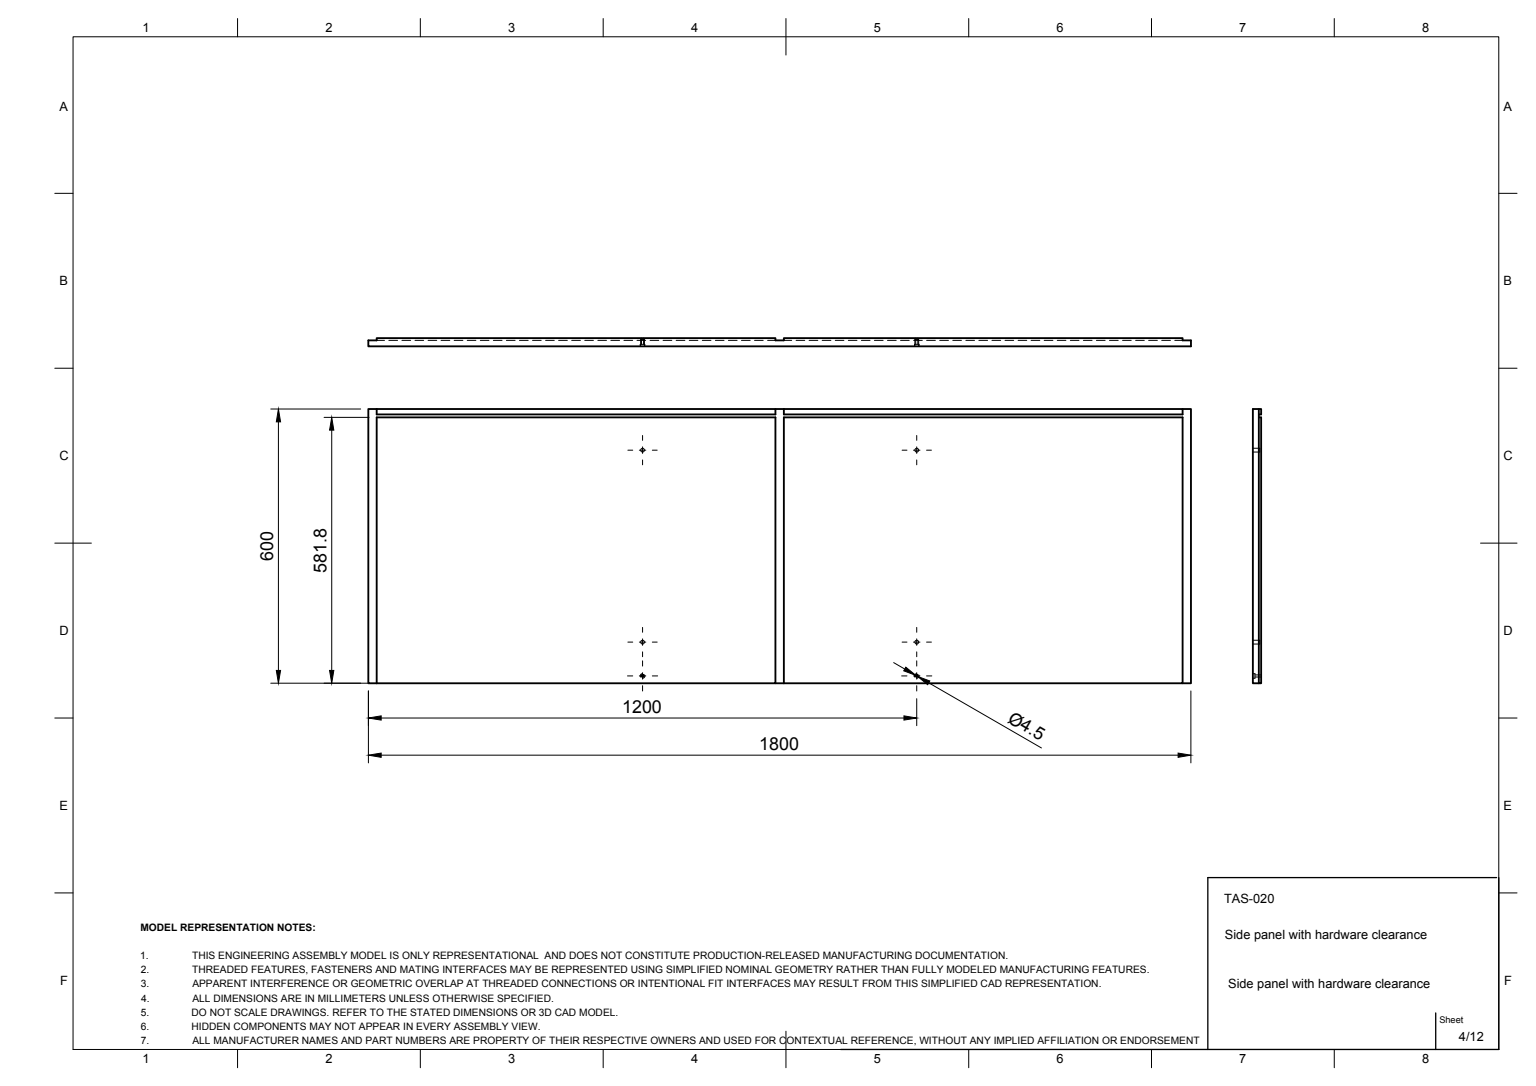
ISO-10303-21;
HEADER;
/* Generated by software containing ST-Developer
 * from STEP Tools, Inc. (www.steptools.com) 
 */

FILE_DESCRIPTION(
/* description */ (''),
/* implementation_level */ '2;1');

FILE_NAME(
/* name */ 'Side panel with hardware clearance.step',
/* time_stamp */ '2026-11-15T17:46:57-08:00',
/* author */ (''),
/* organization */ (''),
/* preprocessor_version */ 'ST-DEVELOPER v20.2',
/* originating_system */ 'Autodesk Translation Framework v15.17.0.0',
/* authorisation */ '');

FILE_SCHEMA (('AUTOMOTIVE_DESIGN { 1 0 10303 214 3 1 1 }'));
ENDSEC;

DATA;
#10=MECHANICAL_DESIGN_GEOMETRIC_PRESENTATION_REPRESENTATION('',(#375),#12963);
#351=SHAPE_REPRESENTATION_RELATIONSHIP('SRR','None',#13035,#363);
#363=ADVANCED_BREP_SHAPE_REPRESENTATION('',(#387),#12951);
#375=STYLED_ITEM('',(#13104),#387);
#387=MANIFOLD_SOLID_BREP('Body1',#4809);
#399=FACE_BOUND('',#830,.T.);
#400=FACE_BOUND('',#833,.T.);
#401=FACE_BOUND('',#852,.T.);
#402=FACE_BOUND('',#859,.T.);
#403=FACE_BOUND('',#867,.T.);
#404=FACE_BOUND('',#868,.T.);
#405=FACE_BOUND('',#869,.T.);
#406=FACE_BOUND('',#870,.T.);
#407=FACE_BOUND('',#871,.T.);
#408=FACE_BOUND('',#872,.T.);
#441=PLANE('',#4959);
#442=PLANE('',#4964);
#443=PLANE('',#4969);
#444=PLANE('',#4973);
#445=PLANE('',#4977);
#446=PLANE('',#4981);
#447=PLANE('',#4986);
#448=PLANE('',#4987);
#449=PLANE('',#4988);
#450=PLANE('',#4989);
#451=PLANE('',#4990);
#452=PLANE('',#4991);
#453=PLANE('',#4992);
#454=PLANE('',#4993);
#455=PLANE('',#4994);
#456=PLANE('',#4995);
#457=PLANE('',#4996);
#458=PLANE('',#4997);
#459=PLANE('',#4998);
#460=PLANE('',#4999);
#461=PLANE('',#5000);
#462=PLANE('',#5001);
#463=PLANE('',#5002);
#464=PLANE('',#5003);
#465=PLANE('',#5004);
#466=PLANE('',#5005);
#467=PLANE('',#5006);
#468=PLANE('',#5007);
#572=FACE_OUTER_BOUND('',#828,.T.);
#573=FACE_OUTER_BOUND('',#829,.T.);
#574=FACE_OUTER_BOUND('',#831,.T.);
#575=FACE_OUTER_BOUND('',#832,.T.);
#576=FACE_OUTER_BOUND('',#834,.T.);
#577=FACE_OUTER_BOUND('',#835,.T.);
#578=FACE_OUTER_BOUND('',#836,.T.);
#579=FACE_OUTER_BOUND('',#837,.T.);
#580=FACE_OUTER_BOUND('',#838,.T.);
#581=FACE_OUTER_BOUND('',#839,.T.);
#582=FACE_OUTER_BOUND('',#840,.T.);
#583=FACE_OUTER_BOUND('',#841,.T.);
#584=FACE_OUTER_BOUND('',#842,.T.);
#585=FACE_OUTER_BOUND('',#843,.T.);
#586=FACE_OUTER_BOUND('',#844,.T.);
#587=FACE_OUTER_BOUND('',#845,.T.);
#588=FACE_OUTER_BOUND('',#846,.T.);
#589=FACE_OUTER_BOUND('',#847,.T.);
#590=FACE_OUTER_BOUND('',#848,.T.);
#591=FACE_OUTER_BOUND('',#849,.T.);
#592=FACE_OUTER_BOUND('',#850,.T.);
#593=FACE_OUTER_BOUND('',#851,.T.);
#594=FACE_OUTER_BOUND('',#853,.T.);
#595=FACE_OUTER_BOUND('',#854,.T.);
#596=FACE_OUTER_BOUND('',#855,.T.);
#597=FACE_OUTER_BOUND('',#856,.T.);
#598=FACE_OUTER_BOUND('',#857,.T.);
#599=FACE_OUTER_BOUND('',#858,.T.);
#600=FACE_OUTER_BOUND('',#860,.T.);
#601=FACE_OUTER_BOUND('',#861,.T.);
#602=FACE_OUTER_BOUND('',#862,.T.);
#603=FACE_OUTER_BOUND('',#863,.T.);
#604=FACE_OUTER_BOUND('',#864,.T.);
#605=FACE_OUTER_BOUND('',#865,.T.);
#606=FACE_OUTER_BOUND('',#866,.T.);
#607=FACE_OUTER_BOUND('',#873,.T.);
#828=EDGE_LOOP('',(#3112,#3113,#3114,#3115));
#829=EDGE_LOOP('',(#3116));
#830=EDGE_LOOP('',(#3117));
#831=EDGE_LOOP('',(#3118,#3119,#3120,#3121));
#832=EDGE_LOOP('',(#3122));
#833=EDGE_LOOP('',(#3123));
#834=EDGE_LOOP('',(#3124,#3125,#3126,#3127));
#835=EDGE_LOOP('',(#3128));
#836=EDGE_LOOP('',(#3129,#3130,#3131,#3132));
#837=EDGE_LOOP('',(#3133));
#838=EDGE_LOOP('',(#3134,#3135,#3136,#3137));
#839=EDGE_LOOP('',(#3138));
#840=EDGE_LOOP('',(#3139,#3140,#3141,#3142));
#841=EDGE_LOOP('',(#3143));
#842=EDGE_LOOP('',(#3144,#3145,#3146,#3147));
#843=EDGE_LOOP('',(#3148,#3149,#3150,#3151));
#844=EDGE_LOOP('',(#3152,#3153,#3154,#3155));
#845=EDGE_LOOP('',(#3156,#3157,#3158,#3159));
#846=EDGE_LOOP('',(#3160,#3161,#3162,#3163));
#847=EDGE_LOOP('',(#3164,#3165,#3166,#3167));
#848=EDGE_LOOP('',(#3168,#3169,#3170,#3171,#3172,#3173,#3174,#3175,#3176,
#3177,#3178,#3179,#3180,#3181,#3182,#3183,#3184,#3185,#3186,#3187));
#849=EDGE_LOOP('',(#3188,#3189,#3190,#3191));
#850=EDGE_LOOP('',(#3192,#3193,#3194,#3195));
#851=EDGE_LOOP('',(#3196,#3197,#3198,#3199));
#852=EDGE_LOOP('',(#3200));
#853=EDGE_LOOP('',(#3201,#3202,#3203,#3204));
#854=EDGE_LOOP('',(#3205,#3206,#3207,#3208));
#855=EDGE_LOOP('',(#3209,#3210,#3211,#3212));
#856=EDGE_LOOP('',(#3213,#3214,#3215,#3216));
#857=EDGE_LOOP('',(#3217,#3218,#3219,#3220));
#858=EDGE_LOOP('',(#3221,#3222,#3223,#3224));
#859=EDGE_LOOP('',(#3225));
#860=EDGE_LOOP('',(#3226,#3227,#3228,#3229));
#861=EDGE_LOOP('',(#3230,#3231,#3232,#3233));
#862=EDGE_LOOP('',(#3234,#3235,#3236,#3237));
#863=EDGE_LOOP('',(#3238,#3239,#3240,#3241,#3242,#3243,#3244,#3245,#3246,
#3247,#3248,#3249));
#864=EDGE_LOOP('',(#3250,#3251,#3252,#3253));
#865=EDGE_LOOP('',(#3254,#3255,#3256,#3257,#3258,#3259,#3260,#3261,#3262,
#3263,#3264,#3265));
#866=EDGE_LOOP('',(#3266,#3267,#3268,#3269));
#867=EDGE_LOOP('',(#3270));
#868=EDGE_LOOP('',(#3271));
#869=EDGE_LOOP('',(#3272));
#870=EDGE_LOOP('',(#3273));
#871=EDGE_LOOP('',(#3274));
#872=EDGE_LOOP('',(#3275));
#873=EDGE_LOOP('',(#3276,#3277,#3278,#3279));
#1126=LINE('',#6523,#1528);
#1127=LINE('',#6532,#1529);
#1128=LINE('',#6541,#1530);
#1129=LINE('',#6548,#1531);
#1130=LINE('',#6555,#1532);
#1131=LINE('',#6562,#1533);
#1132=LINE('',#6568,#1534);
#1133=LINE('',#6572,#1535);
#1134=LINE('',#6576,#1536);
#1135=LINE('',#6578,#1537);
#1136=LINE('',#6580,#1538);
#1137=LINE('',#6581,#1539);
#1138=LINE('',#6585,#1540);
#1139=LINE('',#6587,#1541);
#1140=LINE('',#6589,#1542);
#1141=LINE('',#6590,#1543);
#1142=LINE('',#6594,#1544);
#1143=LINE('',#6596,#1545);
#1144=LINE('',#6598,#1546);
#1145=LINE('',#6599,#1547);
#1146=LINE('',#6603,#1548);
#1147=LINE('',#6605,#1549);
#1148=LINE('',#6607,#1550);
#1149=LINE('',#6608,#1551);
#1150=LINE('',#6611,#1552);
#1151=LINE('',#6613,#1553);
#1152=LINE('',#6615,#1554);
#1153=LINE('',#6617,#1555);
#1154=LINE('',#6618,#1556);
#1155=LINE('',#6620,#1557);
#1156=LINE('',#6622,#1558);
#1157=LINE('',#6623,#1559);
#1158=LINE('',#6625,#1560);
#1159=LINE('',#6627,#1561);
#1160=LINE('',#6629,#1562);
#1161=LINE('',#6631,#1563);
#1162=LINE('',#6632,#1564);
#1163=LINE('',#6634,#1565);
#1164=LINE('',#6636,#1566);
#1165=LINE('',#6637,#1567);
#1166=LINE('',#6640,#1568);
#1167=LINE('',#6641,#1569);
#1168=LINE('',#6644,#1570);
#1169=LINE('',#6645,#1571);
#1170=LINE('',#6648,#1572);
#1171=LINE('',#6649,#1573);
#1172=LINE('',#6652,#1574);
#1173=LINE('',#6653,#1575);
#1174=LINE('',#6655,#1576);
#1175=LINE('',#6657,#1577);
#1176=LINE('',#6660,#1578);
#1177=LINE('',#6661,#1579);
#1178=LINE('',#6664,#1580);
#1179=LINE('',#6665,#1581);
#1180=LINE('',#6668,#1582);
#1181=LINE('',#6669,#1583);
#1182=LINE('',#6672,#1584);
#1183=LINE('',#6673,#1585);
#1184=LINE('',#6675,#1586);
#1185=LINE('',#6677,#1587);
#1186=LINE('',#6680,#1588);
#1187=LINE('',#6682,#1589);
#1188=LINE('',#6683,#1590);
#1189=LINE('',#6686,#1591);
#1190=LINE('',#6687,#1592);
#1191=LINE('',#6690,#1593);
#1192=LINE('',#6691,#1594);
#1193=LINE('',#6693,#1595);
#1528=VECTOR('',#5349,0.5);
#1529=VECTOR('',#5360,0.5);
#1530=VECTOR('',#5371,0.409999999999997);
#1531=VECTOR('',#5380,0.409999999999997);
#1532=VECTOR('',#5389,0.409999999999997);
#1533=VECTOR('',#5398,0.409999999999997);
#1534=VECTOR('',#5407,0.225000000000001);
#1535=VECTOR('',#5412,0.224999999999994);
#1536=VECTOR('',#5415,1.);
#1537=VECTOR('',#5416,1.);
#1538=VECTOR('',#5417,1.);
#1539=VECTOR('',#5418,1.);
#1540=VECTOR('',#5421,1.);
#1541=VECTOR('',#5422,1.);
#1542=VECTOR('',#5423,1.);
#1543=VECTOR('',#5424,1.);
#1544=VECTOR('',#5427,1.);
#1545=VECTOR('',#5428,1.);
#1546=VECTOR('',#5429,1.);
#1547=VECTOR('',#5430,1.);
#1548=VECTOR('',#5433,1.);
#1549=VECTOR('',#5434,1.);
#1550=VECTOR('',#5435,1.);
#1551=VECTOR('',#5436,1.);
#1552=VECTOR('',#5439,1.);
#1553=VECTOR('',#5440,1.);
#1554=VECTOR('',#5441,1.);
#1555=VECTOR('',#5442,1.);
#1556=VECTOR('',#5443,1.);
#1557=VECTOR('',#5444,1.);
#1558=VECTOR('',#5445,1.);
#1559=VECTOR('',#5446,1.);
#1560=VECTOR('',#5447,1.);
#1561=VECTOR('',#5448,1.);
#1562=VECTOR('',#5449,1.);
#1563=VECTOR('',#5450,1.);
#1564=VECTOR('',#5451,1.);
#1565=VECTOR('',#5452,1.);
#1566=VECTOR('',#5453,1.);
#1567=VECTOR('',#5454,1.);
#1568=VECTOR('',#5457,1.);
#1569=VECTOR('',#5458,1.);
#1570=VECTOR('',#5461,1.);
#1571=VECTOR('',#5462,1.);
#1572=VECTOR('',#5465,1.);
#1573=VECTOR('',#5466,1.);
#1574=VECTOR('',#5469,1.);
#1575=VECTOR('',#5470,1.);
#1576=VECTOR('',#5473,1.);
#1577=VECTOR('',#5476,1.);
#1578=VECTOR('',#5479,1.);
#1579=VECTOR('',#5480,1.);
#1580=VECTOR('',#5483,1.);
#1581=VECTOR('',#5484,1.);
#1582=VECTOR('',#5487,1.);
#1583=VECTOR('',#5488,1.);
#1584=VECTOR('',#5491,1.);
#1585=VECTOR('',#5492,1.);
#1586=VECTOR('',#5495,1.);
#1587=VECTOR('',#5498,1.);
#1588=VECTOR('',#5501,1.);
#1589=VECTOR('',#5502,1.);
#1590=VECTOR('',#5503,1.);
#1591=VECTOR('',#5506,1.);
#1592=VECTOR('',#5507,1.);
#1593=VECTOR('',#5510,1.);
#1594=VECTOR('',#5511,1.);
#1595=VECTOR('',#5514,1.);
#1930=CIRCLE('',#4957,0.5);
#1931=CIRCLE('',#4958,0.5);
#1932=CIRCLE('',#4960,0.225000000000001);
#1933=CIRCLE('',#4962,0.5);
#1934=CIRCLE('',#4963,0.5);
#1935=CIRCLE('',#4965,0.224999999999994);
#1936=CIRCLE('',#4967,0.409999999999997);
#1937=CIRCLE('',#4968,0.409999999999997);
#1938=CIRCLE('',#4971,0.409999999999997);
#1939=CIRCLE('',#4972,0.409999999999997);
#1940=CIRCLE('',#4975,0.409999999999997);
#1941=CIRCLE('',#4976,0.409999999999997);
#1942=CIRCLE('',#4979,0.409999999999997);
#1943=CIRCLE('',#4980,0.409999999999997);
#1944=CIRCLE('',#4983,0.225000000000001);
#1945=CIRCLE('',#4985,0.224999999999994);
#2012=VERTEX_POINT('',#6520);
#2013=VERTEX_POINT('',#6522);
#2014=VERTEX_POINT('',#6526);
#2015=VERTEX_POINT('',#6529);
#2016=VERTEX_POINT('',#6531);
#2017=VERTEX_POINT('',#6535);
#2018=VERTEX_POINT('',#6538);
#2019=VERTEX_POINT('',#6540);
#2020=VERTEX_POINT('',#6545);
#2021=VERTEX_POINT('',#6547);
#2022=VERTEX_POINT('',#6552);
#2023=VERTEX_POINT('',#6554);
#2024=VERTEX_POINT('',#6559);
#2025=VERTEX_POINT('',#6561);
#2026=VERTEX_POINT('',#6566);
#2027=VERTEX_POINT('',#6570);
#2028=VERTEX_POINT('',#6574);
#2029=VERTEX_POINT('',#6575);
#2030=VERTEX_POINT('',#6577);
#2031=VERTEX_POINT('',#6579);
#2032=VERTEX_POINT('',#6583);
#2033=VERTEX_POINT('',#6584);
#2034=VERTEX_POINT('',#6586);
#2035=VERTEX_POINT('',#6588);
#2036=VERTEX_POINT('',#6592);
#2037=VERTEX_POINT('',#6593);
#2038=VERTEX_POINT('',#6595);
#2039=VERTEX_POINT('',#6597);
#2040=VERTEX_POINT('',#6601);
#2041=VERTEX_POINT('',#6602);
#2042=VERTEX_POINT('',#6604);
#2043=VERTEX_POINT('',#6606);
#2044=VERTEX_POINT('',#6610);
#2045=VERTEX_POINT('',#6612);
#2046=VERTEX_POINT('',#6614);
#2047=VERTEX_POINT('',#6616);
#2048=VERTEX_POINT('',#6619);
#2049=VERTEX_POINT('',#6621);
#2050=VERTEX_POINT('',#6624);
#2051=VERTEX_POINT('',#6626);
#2052=VERTEX_POINT('',#6628);
#2053=VERTEX_POINT('',#6630);
#2054=VERTEX_POINT('',#6633);
#2055=VERTEX_POINT('',#6635);
#2056=VERTEX_POINT('',#6639);
#2057=VERTEX_POINT('',#6643);
#2058=VERTEX_POINT('',#6647);
#2059=VERTEX_POINT('',#6651);
#2060=VERTEX_POINT('',#6659);
#2061=VERTEX_POINT('',#6663);
#2062=VERTEX_POINT('',#6667);
#2063=VERTEX_POINT('',#6671);
#2064=VERTEX_POINT('',#6679);
#2065=VERTEX_POINT('',#6681);
#2066=VERTEX_POINT('',#6685);
#2067=VERTEX_POINT('',#6689);
#2452=EDGE_CURVE('',#2012,#2012,#1930,.T.);
#2453=EDGE_CURVE('',#2012,#2013,#1126,.T.);
#2454=EDGE_CURVE('',#2013,#2013,#1931,.T.);
#2455=EDGE_CURVE('',#2014,#2014,#1932,.T.);
#2456=EDGE_CURVE('',#2015,#2015,#1933,.T.);
#2457=EDGE_CURVE('',#2015,#2016,#1127,.T.);
#2458=EDGE_CURVE('',#2016,#2016,#1934,.T.);
#2459=EDGE_CURVE('',#2017,#2017,#1935,.T.);
#2460=EDGE_CURVE('',#2018,#2018,#1936,.T.);
#2461=EDGE_CURVE('',#2018,#2019,#1128,.T.);
#2462=EDGE_CURVE('',#2019,#2019,#1937,.T.);
#2463=EDGE_CURVE('',#2020,#2020,#1938,.T.);
#2464=EDGE_CURVE('',#2020,#2021,#1129,.T.);
#2465=EDGE_CURVE('',#2021,#2021,#1939,.T.);
#2466=EDGE_CURVE('',#2022,#2022,#1940,.T.);
#2467=EDGE_CURVE('',#2022,#2023,#1130,.T.);
#2468=EDGE_CURVE('',#2023,#2023,#1941,.T.);
#2469=EDGE_CURVE('',#2024,#2024,#1942,.T.);
#2470=EDGE_CURVE('',#2024,#2025,#1131,.T.);
#2471=EDGE_CURVE('',#2025,#2025,#1943,.T.);
#2472=EDGE_CURVE('',#2026,#2026,#1944,.T.);
#2473=EDGE_CURVE('',#2026,#2014,#1132,.T.);
#2474=EDGE_CURVE('',#2027,#2027,#1945,.T.);
#2475=EDGE_CURVE('',#2027,#2017,#1133,.T.);
#2476=EDGE_CURVE('',#2028,#2029,#1134,.T.);
#2477=EDGE_CURVE('',#2030,#2028,#1135,.T.);
#2478=EDGE_CURVE('',#2031,#2030,#1136,.T.);
#2479=EDGE_CURVE('',#2029,#2031,#1137,.T.);
#2480=EDGE_CURVE('',#2032,#2033,#1138,.T.);
#2481=EDGE_CURVE('',#2034,#2032,#1139,.T.);
#2482=EDGE_CURVE('',#2035,#2034,#1140,.T.);
#2483=EDGE_CURVE('',#2033,#2035,#1141,.T.);
#2484=EDGE_CURVE('',#2036,#2037,#1142,.T.);
#2485=EDGE_CURVE('',#2038,#2036,#1143,.T.);
#2486=EDGE_CURVE('',#2039,#2038,#1144,.T.);
#2487=EDGE_CURVE('',#2039,#2037,#1145,.T.);
#2488=EDGE_CURVE('',#2040,#2041,#1146,.T.);
#2489=EDGE_CURVE('',#2042,#2040,#1147,.T.);
#2490=EDGE_CURVE('',#2043,#2042,#1148,.T.);
#2491=EDGE_CURVE('',#2043,#2041,#1149,.T.);
#2492=EDGE_CURVE('',#2044,#2032,#1150,.T.);
#2493=EDGE_CURVE('',#2045,#2044,#1151,.T.);
#2494=EDGE_CURVE('',#2046,#2045,#1152,.T.);
#2495=EDGE_CURVE('',#2047,#2046,#1153,.T.);
#2496=EDGE_CURVE('',#2041,#2047,#1154,.T.);
#2497=EDGE_CURVE('',#2043,#2048,#1155,.T.);
#2498=EDGE_CURVE('',#2049,#2048,#1156,.T.);
#2499=EDGE_CURVE('',#2037,#2049,#1157,.T.);
#2500=EDGE_CURVE('',#2039,#2050,#1158,.T.);
#2501=EDGE_CURVE('',#2051,#2050,#1159,.T.);
#2502=EDGE_CURVE('',#2052,#2051,#1160,.T.);
#2503=EDGE_CURVE('',#2053,#2052,#1161,.T.);
#2504=EDGE_CURVE('',#2053,#2030,#1162,.T.);
#2505=EDGE_CURVE('',#2054,#2028,#1163,.T.);
#2506=EDGE_CURVE('',#2055,#2054,#1164,.T.);
#2507=EDGE_CURVE('',#2055,#2034,#1165,.T.);
#2508=EDGE_CURVE('',#2056,#2047,#1166,.T.);
#2509=EDGE_CURVE('',#2040,#2056,#1167,.T.);
#2510=EDGE_CURVE('',#2057,#2033,#1168,.T.);
#2511=EDGE_CURVE('',#2044,#2057,#1169,.T.);
#2512=EDGE_CURVE('',#2058,#2056,#1170,.T.);
#2513=EDGE_CURVE('',#2058,#2042,#1171,.T.);
#2514=EDGE_CURVE('',#2035,#2059,#1172,.T.);
#2515=EDGE_CURVE('',#2059,#2057,#1173,.T.);
#2516=EDGE_CURVE('',#2048,#2058,#1174,.T.);
#2517=EDGE_CURVE('',#2059,#2055,#1175,.T.);
#2518=EDGE_CURVE('',#2060,#2049,#1176,.T.);
#2519=EDGE_CURVE('',#2036,#2060,#1177,.T.);
#2520=EDGE_CURVE('',#2061,#2029,#1178,.T.);
#2521=EDGE_CURVE('',#2054,#2061,#1179,.T.);
#2522=EDGE_CURVE('',#2062,#2060,#1180,.T.);
#2523=EDGE_CURVE('',#2062,#2038,#1181,.T.);
#2524=EDGE_CURVE('',#2031,#2063,#1182,.T.);
#2525=EDGE_CURVE('',#2063,#2061,#1183,.T.);
#2526=EDGE_CURVE('',#2050,#2062,#1184,.T.);
#2527=EDGE_CURVE('',#2063,#2053,#1185,.T.);
#2528=EDGE_CURVE('',#2052,#2064,#1186,.T.);
#2529=EDGE_CURVE('',#2064,#2065,#1187,.T.);
#2530=EDGE_CURVE('',#2045,#2065,#1188,.T.);
#2531=EDGE_CURVE('',#2066,#2051,#1189,.T.);
#2532=EDGE_CURVE('',#2064,#2066,#1190,.T.);
#2533=EDGE_CURVE('',#2067,#2046,#1191,.T.);
#2534=EDGE_CURVE('',#2066,#2067,#1192,.T.);
#2535=EDGE_CURVE('',#2065,#2067,#1193,.T.);
#3112=ORIENTED_EDGE('',*,*,#2452,.F.);
#3113=ORIENTED_EDGE('',*,*,#2453,.T.);
#3114=ORIENTED_EDGE('',*,*,#2454,.T.);
#3115=ORIENTED_EDGE('',*,*,#2453,.F.);
#3116=ORIENTED_EDGE('',*,*,#2454,.F.);
#3117=ORIENTED_EDGE('',*,*,#2455,.F.);
#3118=ORIENTED_EDGE('',*,*,#2456,.F.);
#3119=ORIENTED_EDGE('',*,*,#2457,.T.);
#3120=ORIENTED_EDGE('',*,*,#2458,.T.);
#3121=ORIENTED_EDGE('',*,*,#2457,.F.);
#3122=ORIENTED_EDGE('',*,*,#2458,.F.);
#3123=ORIENTED_EDGE('',*,*,#2459,.F.);
#3124=ORIENTED_EDGE('',*,*,#2460,.F.);
#3125=ORIENTED_EDGE('',*,*,#2461,.T.);
#3126=ORIENTED_EDGE('',*,*,#2462,.T.);
#3127=ORIENTED_EDGE('',*,*,#2461,.F.);
#3128=ORIENTED_EDGE('',*,*,#2462,.F.);
#3129=ORIENTED_EDGE('',*,*,#2463,.F.);
#3130=ORIENTED_EDGE('',*,*,#2464,.T.);
#3131=ORIENTED_EDGE('',*,*,#2465,.T.);
#3132=ORIENTED_EDGE('',*,*,#2464,.F.);
#3133=ORIENTED_EDGE('',*,*,#2465,.F.);
#3134=ORIENTED_EDGE('',*,*,#2466,.F.);
#3135=ORIENTED_EDGE('',*,*,#2467,.T.);
#3136=ORIENTED_EDGE('',*,*,#2468,.T.);
#3137=ORIENTED_EDGE('',*,*,#2467,.F.);
#3138=ORIENTED_EDGE('',*,*,#2468,.F.);
#3139=ORIENTED_EDGE('',*,*,#2469,.F.);
#3140=ORIENTED_EDGE('',*,*,#2470,.T.);
#3141=ORIENTED_EDGE('',*,*,#2471,.T.);
#3142=ORIENTED_EDGE('',*,*,#2470,.F.);
#3143=ORIENTED_EDGE('',*,*,#2471,.F.);
#3144=ORIENTED_EDGE('',*,*,#2472,.F.);
#3145=ORIENTED_EDGE('',*,*,#2473,.T.);
#3146=ORIENTED_EDGE('',*,*,#2455,.T.);
#3147=ORIENTED_EDGE('',*,*,#2473,.F.);
#3148=ORIENTED_EDGE('',*,*,#2474,.F.);
#3149=ORIENTED_EDGE('',*,*,#2475,.T.);
#3150=ORIENTED_EDGE('',*,*,#2459,.T.);
#3151=ORIENTED_EDGE('',*,*,#2475,.F.);
#3152=ORIENTED_EDGE('',*,*,#2476,.F.);
#3153=ORIENTED_EDGE('',*,*,#2477,.F.);
#3154=ORIENTED_EDGE('',*,*,#2478,.F.);
#3155=ORIENTED_EDGE('',*,*,#2479,.F.);
#3156=ORIENTED_EDGE('',*,*,#2480,.F.);
#3157=ORIENTED_EDGE('',*,*,#2481,.F.);
#3158=ORIENTED_EDGE('',*,*,#2482,.F.);
#3159=ORIENTED_EDGE('',*,*,#2483,.F.);
#3160=ORIENTED_EDGE('',*,*,#2484,.F.);
#3161=ORIENTED_EDGE('',*,*,#2485,.F.);
#3162=ORIENTED_EDGE('',*,*,#2486,.F.);
#3163=ORIENTED_EDGE('',*,*,#2487,.T.);
#3164=ORIENTED_EDGE('',*,*,#2488,.F.);
#3165=ORIENTED_EDGE('',*,*,#2489,.F.);
#3166=ORIENTED_EDGE('',*,*,#2490,.F.);
#3167=ORIENTED_EDGE('',*,*,#2491,.T.);
#3168=ORIENTED_EDGE('',*,*,#2492,.F.);
#3169=ORIENTED_EDGE('',*,*,#2493,.F.);
#3170=ORIENTED_EDGE('',*,*,#2494,.F.);
#3171=ORIENTED_EDGE('',*,*,#2495,.F.);
#3172=ORIENTED_EDGE('',*,*,#2496,.F.);
#3173=ORIENTED_EDGE('',*,*,#2491,.F.);
#3174=ORIENTED_EDGE('',*,*,#2497,.T.);
#3175=ORIENTED_EDGE('',*,*,#2498,.F.);
#3176=ORIENTED_EDGE('',*,*,#2499,.F.);
#3177=ORIENTED_EDGE('',*,*,#2487,.F.);
#3178=ORIENTED_EDGE('',*,*,#2500,.T.);
#3179=ORIENTED_EDGE('',*,*,#2501,.F.);
#3180=ORIENTED_EDGE('',*,*,#2502,.F.);
#3181=ORIENTED_EDGE('',*,*,#2503,.F.);
#3182=ORIENTED_EDGE('',*,*,#2504,.T.);
#3183=ORIENTED_EDGE('',*,*,#2477,.T.);
#3184=ORIENTED_EDGE('',*,*,#2505,.F.);
#3185=ORIENTED_EDGE('',*,*,#2506,.F.);
#3186=ORIENTED_EDGE('',*,*,#2507,.T.);
#3187=ORIENTED_EDGE('',*,*,#2481,.T.);
#3188=ORIENTED_EDGE('',*,*,#2488,.T.);
#3189=ORIENTED_EDGE('',*,*,#2496,.T.);
#3190=ORIENTED_EDGE('',*,*,#2508,.F.);
#3191=ORIENTED_EDGE('',*,*,#2509,.F.);
#3192=ORIENTED_EDGE('',*,*,#2480,.T.);
#3193=ORIENTED_EDGE('',*,*,#2510,.F.);
#3194=ORIENTED_EDGE('',*,*,#2511,.F.);
#3195=ORIENTED_EDGE('',*,*,#2492,.T.);
#3196=ORIENTED_EDGE('',*,*,#2489,.T.);
#3197=ORIENTED_EDGE('',*,*,#2509,.T.);
#3198=ORIENTED_EDGE('',*,*,#2512,.F.);
#3199=ORIENTED_EDGE('',*,*,#2513,.T.);
#3200=ORIENTED_EDGE('',*,*,#2474,.T.);
#3201=ORIENTED_EDGE('',*,*,#2483,.T.);
#3202=ORIENTED_EDGE('',*,*,#2514,.T.);
#3203=ORIENTED_EDGE('',*,*,#2515,.T.);
#3204=ORIENTED_EDGE('',*,*,#2510,.T.);
#3205=ORIENTED_EDGE('',*,*,#2490,.T.);
#3206=ORIENTED_EDGE('',*,*,#2513,.F.);
#3207=ORIENTED_EDGE('',*,*,#2516,.F.);
#3208=ORIENTED_EDGE('',*,*,#2497,.F.);
#3209=ORIENTED_EDGE('',*,*,#2482,.T.);
#3210=ORIENTED_EDGE('',*,*,#2507,.F.);
#3211=ORIENTED_EDGE('',*,*,#2517,.F.);
#3212=ORIENTED_EDGE('',*,*,#2514,.F.);
#3213=ORIENTED_EDGE('',*,*,#2484,.T.);
#3214=ORIENTED_EDGE('',*,*,#2499,.T.);
#3215=ORIENTED_EDGE('',*,*,#2518,.F.);
#3216=ORIENTED_EDGE('',*,*,#2519,.F.);
#3217=ORIENTED_EDGE('',*,*,#2476,.T.);
#3218=ORIENTED_EDGE('',*,*,#2520,.F.);
#3219=ORIENTED_EDGE('',*,*,#2521,.F.);
#3220=ORIENTED_EDGE('',*,*,#2505,.T.);
#3221=ORIENTED_EDGE('',*,*,#2485,.T.);
#3222=ORIENTED_EDGE('',*,*,#2519,.T.);
#3223=ORIENTED_EDGE('',*,*,#2522,.F.);
#3224=ORIENTED_EDGE('',*,*,#2523,.T.);
#3225=ORIENTED_EDGE('',*,*,#2472,.T.);
#3226=ORIENTED_EDGE('',*,*,#2479,.T.);
#3227=ORIENTED_EDGE('',*,*,#2524,.T.);
#3228=ORIENTED_EDGE('',*,*,#2525,.T.);
#3229=ORIENTED_EDGE('',*,*,#2520,.T.);
#3230=ORIENTED_EDGE('',*,*,#2486,.T.);
#3231=ORIENTED_EDGE('',*,*,#2523,.F.);
#3232=ORIENTED_EDGE('',*,*,#2526,.F.);
#3233=ORIENTED_EDGE('',*,*,#2500,.F.);
#3234=ORIENTED_EDGE('',*,*,#2478,.T.);
#3235=ORIENTED_EDGE('',*,*,#2504,.F.);
#3236=ORIENTED_EDGE('',*,*,#2527,.F.);
#3237=ORIENTED_EDGE('',*,*,#2524,.F.);
#3238=ORIENTED_EDGE('',*,*,#2517,.T.);
#3239=ORIENTED_EDGE('',*,*,#2506,.T.);
#3240=ORIENTED_EDGE('',*,*,#2521,.T.);
#3241=ORIENTED_EDGE('',*,*,#2525,.F.);
#3242=ORIENTED_EDGE('',*,*,#2527,.T.);
#3243=ORIENTED_EDGE('',*,*,#2503,.T.);
#3244=ORIENTED_EDGE('',*,*,#2528,.T.);
#3245=ORIENTED_EDGE('',*,*,#2529,.T.);
#3246=ORIENTED_EDGE('',*,*,#2530,.F.);
#3247=ORIENTED_EDGE('',*,*,#2493,.T.);
#3248=ORIENTED_EDGE('',*,*,#2511,.T.);
#3249=ORIENTED_EDGE('',*,*,#2515,.F.);
#3250=ORIENTED_EDGE('',*,*,#2502,.T.);
#3251=ORIENTED_EDGE('',*,*,#2531,.F.);
#3252=ORIENTED_EDGE('',*,*,#2532,.F.);
#3253=ORIENTED_EDGE('',*,*,#2528,.F.);
#3254=ORIENTED_EDGE('',*,*,#2516,.T.);
#3255=ORIENTED_EDGE('',*,*,#2512,.T.);
#3256=ORIENTED_EDGE('',*,*,#2508,.T.);
#3257=ORIENTED_EDGE('',*,*,#2495,.T.);
#3258=ORIENTED_EDGE('',*,*,#2533,.F.);
#3259=ORIENTED_EDGE('',*,*,#2534,.F.);
#3260=ORIENTED_EDGE('',*,*,#2531,.T.);
#3261=ORIENTED_EDGE('',*,*,#2501,.T.);
#3262=ORIENTED_EDGE('',*,*,#2526,.T.);
#3263=ORIENTED_EDGE('',*,*,#2522,.T.);
#3264=ORIENTED_EDGE('',*,*,#2518,.T.);
#3265=ORIENTED_EDGE('',*,*,#2498,.T.);
#3266=ORIENTED_EDGE('',*,*,#2532,.T.);
#3267=ORIENTED_EDGE('',*,*,#2534,.T.);
#3268=ORIENTED_EDGE('',*,*,#2535,.F.);
#3269=ORIENTED_EDGE('',*,*,#2529,.F.);
#3270=ORIENTED_EDGE('',*,*,#2460,.T.);
#3271=ORIENTED_EDGE('',*,*,#2463,.T.);
#3272=ORIENTED_EDGE('',*,*,#2466,.T.);
#3273=ORIENTED_EDGE('',*,*,#2469,.T.);
#3274=ORIENTED_EDGE('',*,*,#2456,.T.);
#3275=ORIENTED_EDGE('',*,*,#2452,.T.);
#3276=ORIENTED_EDGE('',*,*,#2494,.T.);
#3277=ORIENTED_EDGE('',*,*,#2530,.T.);
#3278=ORIENTED_EDGE('',*,*,#2535,.T.);
#3279=ORIENTED_EDGE('',*,*,#2533,.T.);
#4432=CYLINDRICAL_SURFACE('',#4956,0.5);
#4433=CYLINDRICAL_SURFACE('',#4961,0.5);
#4434=CYLINDRICAL_SURFACE('',#4966,0.409999999999997);
#4435=CYLINDRICAL_SURFACE('',#4970,0.409999999999997);
#4436=CYLINDRICAL_SURFACE('',#4974,0.409999999999997);
#4437=CYLINDRICAL_SURFACE('',#4978,0.409999999999997);
#4438=CYLINDRICAL_SURFACE('',#4982,0.225000000000001);
#4439=CYLINDRICAL_SURFACE('',#4984,0.224999999999994);
#4553=ADVANCED_FACE('',(#572),#4432,.F.);
#4554=ADVANCED_FACE('',(#573,#399),#441,.F.);
#4555=ADVANCED_FACE('',(#574),#4433,.F.);
#4556=ADVANCED_FACE('',(#575,#400),#442,.F.);
#4557=ADVANCED_FACE('',(#576),#4434,.F.);
#4558=ADVANCED_FACE('',(#577),#443,.F.);
#4559=ADVANCED_FACE('',(#578),#4435,.F.);
#4560=ADVANCED_FACE('',(#579),#444,.F.);
#4561=ADVANCED_FACE('',(#580),#4436,.F.);
#4562=ADVANCED_FACE('',(#581),#445,.F.);
#4563=ADVANCED_FACE('',(#582),#4437,.F.);
#4564=ADVANCED_FACE('',(#583),#446,.F.);
#4565=ADVANCED_FACE('',(#584),#4438,.F.);
#4566=ADVANCED_FACE('',(#585),#4439,.F.);
#4567=ADVANCED_FACE('',(#586),#447,.F.);
#4568=ADVANCED_FACE('',(#587),#448,.F.);
#4569=ADVANCED_FACE('',(#588),#449,.F.);
#4570=ADVANCED_FACE('',(#589),#450,.F.);
#4571=ADVANCED_FACE('',(#590),#451,.F.);
#4572=ADVANCED_FACE('',(#591),#452,.T.);
#4573=ADVANCED_FACE('',(#592),#453,.T.);
#4574=ADVANCED_FACE('',(#593,#401),#454,.T.);
#4575=ADVANCED_FACE('',(#594),#455,.T.);
#4576=ADVANCED_FACE('',(#595),#456,.F.);
#4577=ADVANCED_FACE('',(#596),#457,.F.);
#4578=ADVANCED_FACE('',(#597),#458,.T.);
#4579=ADVANCED_FACE('',(#598),#459,.T.);
#4580=ADVANCED_FACE('',(#599,#402),#460,.T.);
#4581=ADVANCED_FACE('',(#600),#461,.T.);
#4582=ADVANCED_FACE('',(#601),#462,.F.);
#4583=ADVANCED_FACE('',(#602),#463,.F.);
#4584=ADVANCED_FACE('',(#603),#464,.T.);
#4585=ADVANCED_FACE('',(#604),#465,.F.);
#4586=ADVANCED_FACE('',(#605),#466,.T.);
#4587=ADVANCED_FACE('',(#606,#403,#404,#405,#406,#407,#408),#467,.T.);
#4588=ADVANCED_FACE('',(#607),#468,.T.);
#4809=CLOSED_SHELL('',(#4553,#4554,#4555,#4556,#4557,#4558,#4559,#4560,
#4561,#4562,#4563,#4564,#4565,#4566,#4567,#4568,#4569,#4570,#4571,#4572,
#4573,#4574,#4575,#4576,#4577,#4578,#4579,#4580,#4581,#4582,#4583,#4584,
#4585,#4586,#4587,#4588));
#4955=AXIS2_PLACEMENT_3D('',#6518,#5343,#5344);
#4956=AXIS2_PLACEMENT_3D('',#6519,#5345,#5346);
#4957=AXIS2_PLACEMENT_3D('',#6521,#5347,#5348);
#4958=AXIS2_PLACEMENT_3D('',#6524,#5350,#5351);
#4959=AXIS2_PLACEMENT_3D('',#6525,#5352,#5353);
#4960=AXIS2_PLACEMENT_3D('',#6527,#5354,#5355);
#4961=AXIS2_PLACEMENT_3D('',#6528,#5356,#5357);
#4962=AXIS2_PLACEMENT_3D('',#6530,#5358,#5359);
#4963=AXIS2_PLACEMENT_3D('',#6533,#5361,#5362);
#4964=AXIS2_PLACEMENT_3D('',#6534,#5363,#5364);
#4965=AXIS2_PLACEMENT_3D('',#6536,#5365,#5366);
#4966=AXIS2_PLACEMENT_3D('',#6537,#5367,#5368);
#4967=AXIS2_PLACEMENT_3D('',#6539,#5369,#5370);
#4968=AXIS2_PLACEMENT_3D('',#6542,#5372,#5373);
#4969=AXIS2_PLACEMENT_3D('',#6543,#5374,#5375);
#4970=AXIS2_PLACEMENT_3D('',#6544,#5376,#5377);
#4971=AXIS2_PLACEMENT_3D('',#6546,#5378,#5379);
#4972=AXIS2_PLACEMENT_3D('',#6549,#5381,#5382);
#4973=AXIS2_PLACEMENT_3D('',#6550,#5383,#5384);
#4974=AXIS2_PLACEMENT_3D('',#6551,#5385,#5386);
#4975=AXIS2_PLACEMENT_3D('',#6553,#5387,#5388);
#4976=AXIS2_PLACEMENT_3D('',#6556,#5390,#5391);
#4977=AXIS2_PLACEMENT_3D('',#6557,#5392,#5393);
#4978=AXIS2_PLACEMENT_3D('',#6558,#5394,#5395);
#4979=AXIS2_PLACEMENT_3D('',#6560,#5396,#5397);
#4980=AXIS2_PLACEMENT_3D('',#6563,#5399,#5400);
#4981=AXIS2_PLACEMENT_3D('',#6564,#5401,#5402);
#4982=AXIS2_PLACEMENT_3D('',#6565,#5403,#5404);
#4983=AXIS2_PLACEMENT_3D('',#6567,#5405,#5406);
#4984=AXIS2_PLACEMENT_3D('',#6569,#5408,#5409);
#4985=AXIS2_PLACEMENT_3D('',#6571,#5410,#5411);
#4986=AXIS2_PLACEMENT_3D('',#6573,#5413,#5414);
#4987=AXIS2_PLACEMENT_3D('',#6582,#5419,#5420);
#4988=AXIS2_PLACEMENT_3D('',#6591,#5425,#5426);
#4989=AXIS2_PLACEMENT_3D('',#6600,#5431,#5432);
#4990=AXIS2_PLACEMENT_3D('',#6609,#5437,#5438);
#4991=AXIS2_PLACEMENT_3D('',#6638,#5455,#5456);
#4992=AXIS2_PLACEMENT_3D('',#6642,#5459,#5460);
#4993=AXIS2_PLACEMENT_3D('',#6646,#5463,#5464);
#4994=AXIS2_PLACEMENT_3D('',#6650,#5467,#5468);
#4995=AXIS2_PLACEMENT_3D('',#6654,#5471,#5472);
#4996=AXIS2_PLACEMENT_3D('',#6656,#5474,#5475);
#4997=AXIS2_PLACEMENT_3D('',#6658,#5477,#5478);
#4998=AXIS2_PLACEMENT_3D('',#6662,#5481,#5482);
#4999=AXIS2_PLACEMENT_3D('',#6666,#5485,#5486);
#5000=AXIS2_PLACEMENT_3D('',#6670,#5489,#5490);
#5001=AXIS2_PLACEMENT_3D('',#6674,#5493,#5494);
#5002=AXIS2_PLACEMENT_3D('',#6676,#5496,#5497);
#5003=AXIS2_PLACEMENT_3D('',#6678,#5499,#5500);
#5004=AXIS2_PLACEMENT_3D('',#6684,#5504,#5505);
#5005=AXIS2_PLACEMENT_3D('',#6688,#5508,#5509);
#5006=AXIS2_PLACEMENT_3D('',#6692,#5512,#5513);
#5007=AXIS2_PLACEMENT_3D('',#6694,#5515,#5516);
#5343=DIRECTION('axis',(0.,0.,1.));
#5344=DIRECTION('refdir',(1.,0.,0.));
#5345=DIRECTION('center_axis',(1.,0.,0.));
#5346=DIRECTION('ref_axis',(0.,0.,-1.));
#5347=DIRECTION('center_axis',(1.,0.,0.));
#5348=DIRECTION('ref_axis',(0.,0.,-1.));
#5349=DIRECTION('',(1.,0.,0.));
#5350=DIRECTION('center_axis',(1.,0.,0.));
#5351=DIRECTION('ref_axis',(0.,0.,-1.));
#5352=DIRECTION('center_axis',(1.,0.,0.));
#5353=DIRECTION('ref_axis',(0.,0.,-1.));
#5354=DIRECTION('center_axis',(-1.,0.,0.));
#5355=DIRECTION('ref_axis',(0.,0.,-1.));
#5356=DIRECTION('center_axis',(1.,0.,0.));
#5357=DIRECTION('ref_axis',(0.,0.,-1.));
#5358=DIRECTION('center_axis',(1.,0.,0.));
#5359=DIRECTION('ref_axis',(0.,0.,-1.));
#5360=DIRECTION('',(1.,0.,0.));
#5361=DIRECTION('center_axis',(1.,0.,0.));
#5362=DIRECTION('ref_axis',(0.,0.,-1.));
#5363=DIRECTION('center_axis',(1.,0.,0.));
#5364=DIRECTION('ref_axis',(0.,0.,-1.));
#5365=DIRECTION('center_axis',(-1.,0.,0.));
#5366=DIRECTION('ref_axis',(0.,0.,-1.));
#5367=DIRECTION('center_axis',(1.,0.,0.));
#5368=DIRECTION('ref_axis',(0.,0.,-1.));
#5369=DIRECTION('center_axis',(1.,0.,0.));
#5370=DIRECTION('ref_axis',(0.,0.,-1.));
#5371=DIRECTION('',(1.,0.,0.));
#5372=DIRECTION('center_axis',(1.,0.,0.));
#5373=DIRECTION('ref_axis',(0.,0.,-1.));
#5374=DIRECTION('center_axis',(1.,0.,0.));
#5375=DIRECTION('ref_axis',(0.,0.,-1.));
#5376=DIRECTION('center_axis',(1.,0.,0.));
#5377=DIRECTION('ref_axis',(0.,0.,-1.));
#5378=DIRECTION('center_axis',(1.,0.,0.));
#5379=DIRECTION('ref_axis',(0.,0.,-1.));
#5380=DIRECTION('',(1.,0.,0.));
#5381=DIRECTION('center_axis',(1.,0.,0.));
#5382=DIRECTION('ref_axis',(0.,0.,-1.));
#5383=DIRECTION('center_axis',(1.,0.,0.));
#5384=DIRECTION('ref_axis',(0.,0.,-1.));
#5385=DIRECTION('center_axis',(1.,0.,0.));
#5386=DIRECTION('ref_axis',(0.,0.,-1.));
#5387=DIRECTION('center_axis',(1.,0.,0.));
#5388=DIRECTION('ref_axis',(0.,0.,-1.));
#5389=DIRECTION('',(1.,0.,0.));
#5390=DIRECTION('center_axis',(1.,0.,0.));
#5391=DIRECTION('ref_axis',(0.,0.,-1.));
#5392=DIRECTION('center_axis',(1.,0.,0.));
#5393=DIRECTION('ref_axis',(0.,0.,-1.));
#5394=DIRECTION('center_axis',(1.,0.,0.));
#5395=DIRECTION('ref_axis',(0.,0.,-1.));
#5396=DIRECTION('center_axis',(1.,0.,0.));
#5397=DIRECTION('ref_axis',(0.,0.,-1.));
#5398=DIRECTION('',(1.,0.,0.));
#5399=DIRECTION('center_axis',(1.,0.,0.));
#5400=DIRECTION('ref_axis',(0.,0.,-1.));
#5401=DIRECTION('center_axis',(1.,0.,0.));
#5402=DIRECTION('ref_axis',(0.,0.,-1.));
#5403=DIRECTION('center_axis',(-1.,0.,0.));
#5404=DIRECTION('ref_axis',(0.,0.,-1.));
#5405=DIRECTION('center_axis',(-1.,0.,0.));
#5406=DIRECTION('ref_axis',(0.,0.,-1.));
#5407=DIRECTION('',(-1.,0.,0.));
#5408=DIRECTION('center_axis',(-1.,0.,0.));
#5409=DIRECTION('ref_axis',(0.,0.,-1.));
#5410=DIRECTION('center_axis',(-1.,0.,0.));
#5411=DIRECTION('ref_axis',(0.,0.,-1.));
#5412=DIRECTION('',(-1.,0.,0.));
#5413=DIRECTION('center_axis',(0.,1.,0.));
#5414=DIRECTION('ref_axis',(-1.,0.,0.));
#5415=DIRECTION('',(1.,0.,0.));
#5416=DIRECTION('',(0.,0.,1.));
#5417=DIRECTION('',(-1.,0.,0.));
#5418=DIRECTION('',(0.,0.,-1.));
#5419=DIRECTION('center_axis',(0.,1.,0.));
#5420=DIRECTION('ref_axis',(-1.,0.,0.));
#5421=DIRECTION('',(1.,0.,0.));
#5422=DIRECTION('',(0.,0.,1.));
#5423=DIRECTION('',(-1.,0.,0.));
#5424=DIRECTION('',(0.,0.,-1.));
#5425=DIRECTION('center_axis',(0.,-1.,0.));
#5426=DIRECTION('ref_axis',(1.,0.,0.));
#5427=DIRECTION('',(-1.,0.,0.));
#5428=DIRECTION('',(0.,0.,1.));
#5429=DIRECTION('',(1.,0.,0.));
#5430=DIRECTION('',(0.,0.,1.));
#5431=DIRECTION('center_axis',(0.,-1.,0.));
#5432=DIRECTION('ref_axis',(1.,0.,0.));
#5433=DIRECTION('',(-1.,0.,0.));
#5434=DIRECTION('',(0.,0.,1.));
#5435=DIRECTION('',(1.,0.,0.));
#5436=DIRECTION('',(0.,0.,1.));
#5437=DIRECTION('center_axis',(-1.,0.,0.));
#5438=DIRECTION('ref_axis',(0.,-1.,0.));
#5439=DIRECTION('',(0.,-1.,0.));
#5440=DIRECTION('',(0.,0.,-1.));
#5441=DIRECTION('',(0.,1.,0.));
#5442=DIRECTION('',(0.,0.,1.));
#5443=DIRECTION('',(0.,-1.,0.));
#5444=DIRECTION('',(0.,-1.,0.));
#5445=DIRECTION('',(0.,0.,1.));
#5446=DIRECTION('',(0.,-1.,0.));
#5447=DIRECTION('',(0.,-1.,0.));
#5448=DIRECTION('',(0.,0.,1.));
#5449=DIRECTION('',(0.,-1.,0.));
#5450=DIRECTION('',(0.,0.,-1.));
#5451=DIRECTION('',(0.,-1.,0.));
#5452=DIRECTION('',(0.,-1.,0.));
#5453=DIRECTION('',(0.,0.,-1.));
#5454=DIRECTION('',(0.,-1.,0.));
#5455=DIRECTION('center_axis',(0.,0.,1.));
#5456=DIRECTION('ref_axis',(1.,0.,0.));
#5457=DIRECTION('',(-1.,0.,0.));
#5458=DIRECTION('',(0.,-1.,0.));
#5459=DIRECTION('center_axis',(0.,0.,1.));
#5460=DIRECTION('ref_axis',(1.,0.,0.));
#5461=DIRECTION('',(0.,-1.,0.));
#5462=DIRECTION('',(1.,0.,0.));
#5463=DIRECTION('center_axis',(1.,0.,0.));
#5464=DIRECTION('ref_axis',(0.,1.,0.));
#5465=DIRECTION('',(0.,0.,1.));
#5466=DIRECTION('',(0.,1.,0.));
#5467=DIRECTION('center_axis',(1.,0.,0.));
#5468=DIRECTION('ref_axis',(0.,1.,0.));
#5469=DIRECTION('',(0.,1.,0.));
#5470=DIRECTION('',(0.,0.,1.));
#5471=DIRECTION('center_axis',(0.,0.,1.));
#5472=DIRECTION('ref_axis',(1.,0.,0.));
#5473=DIRECTION('',(1.,0.,0.));
#5474=DIRECTION('center_axis',(0.,0.,1.));
#5475=DIRECTION('ref_axis',(1.,0.,0.));
#5476=DIRECTION('',(-1.,0.,0.));
#5477=DIRECTION('center_axis',(0.,0.,1.));
#5478=DIRECTION('ref_axis',(1.,0.,0.));
#5479=DIRECTION('',(-1.,0.,0.));
#5480=DIRECTION('',(0.,-1.,0.));
#5481=DIRECTION('center_axis',(0.,0.,1.));
#5482=DIRECTION('ref_axis',(1.,0.,0.));
#5483=DIRECTION('',(0.,-1.,0.));
#5484=DIRECTION('',(1.,0.,0.));
#5485=DIRECTION('center_axis',(1.,0.,0.));
#5486=DIRECTION('ref_axis',(0.,1.,0.));
#5487=DIRECTION('',(0.,0.,1.));
#5488=DIRECTION('',(0.,1.,0.));
#5489=DIRECTION('center_axis',(1.,0.,0.));
#5490=DIRECTION('ref_axis',(0.,1.,0.));
#5491=DIRECTION('',(0.,1.,0.));
#5492=DIRECTION('',(0.,0.,1.));
#5493=DIRECTION('center_axis',(0.,0.,1.));
#5494=DIRECTION('ref_axis',(1.,0.,0.));
#5495=DIRECTION('',(1.,0.,0.));
#5496=DIRECTION('center_axis',(0.,0.,1.));
#5497=DIRECTION('ref_axis',(1.,0.,0.));
#5498=DIRECTION('',(-1.,0.,0.));
#5499=DIRECTION('center_axis',(0.,1.,0.));
#5500=DIRECTION('ref_axis',(-1.,0.,0.));
#5501=DIRECTION('',(-1.,0.,0.));
#5502=DIRECTION('',(0.,0.,1.));
#5503=DIRECTION('',(-1.,0.,0.));
#5504=DIRECTION('center_axis',(0.,0.,1.));
#5505=DIRECTION('ref_axis',(1.,0.,0.));
#5506=DIRECTION('',(1.,0.,0.));
#5507=DIRECTION('',(0.,-1.,0.));
#5508=DIRECTION('center_axis',(0.,-1.,0.));
#5509=DIRECTION('ref_axis',(1.,0.,0.));
#5510=DIRECTION('',(1.,0.,0.));
#5511=DIRECTION('',(0.,0.,1.));
#5512=DIRECTION('center_axis',(-1.,0.,0.));
#5513=DIRECTION('ref_axis',(0.,-1.,0.));
#5514=DIRECTION('',(0.,-1.,0.));
#5515=DIRECTION('center_axis',(0.,0.,1.));
#5516=DIRECTION('ref_axis',(1.,0.,0.));
#6518=CARTESIAN_POINT('',(0.,0.,0.));
#6519=CARTESIAN_POINT('Origin',(0.,1.6,60.));
#6520=CARTESIAN_POINT('',(0.,1.6,60.5));
#6521=CARTESIAN_POINT('Origin',(0.,1.6,60.));
#6522=CARTESIAN_POINT('',(0.45,1.6,60.5));
#6523=CARTESIAN_POINT('',(0.,1.6,60.5));
#6524=CARTESIAN_POINT('Origin',(0.45,1.6,60.));
#6525=CARTESIAN_POINT('Origin',(0.45,1.6,60.));
#6526=CARTESIAN_POINT('',(0.45,1.6,60.225));
#6527=CARTESIAN_POINT('Origin',(0.45,1.6,60.));
#6528=CARTESIAN_POINT('Origin',(0.,1.6,120.));
#6529=CARTESIAN_POINT('',(0.,1.6,120.5));
#6530=CARTESIAN_POINT('Origin',(0.,1.6,120.));
#6531=CARTESIAN_POINT('',(0.45,1.6,120.5));
#6532=CARTESIAN_POINT('',(0.,1.6,120.5));
#6533=CARTESIAN_POINT('Origin',(0.45,1.6,120.));
#6534=CARTESIAN_POINT('Origin',(0.45,1.6,120.));
#6535=CARTESIAN_POINT('',(0.45,1.6,120.225));
#6536=CARTESIAN_POINT('Origin',(0.45,1.6,120.));
#6537=CARTESIAN_POINT('Origin',(0.,51.,60.));
#6538=CARTESIAN_POINT('',(0.,51.,60.41));
#6539=CARTESIAN_POINT('Origin',(0.,51.,60.));
#6540=CARTESIAN_POINT('',(1.5,51.,60.41));
#6541=CARTESIAN_POINT('',(0.,51.,60.41));
#6542=CARTESIAN_POINT('Origin',(1.5,51.,60.));
#6543=CARTESIAN_POINT('Origin',(1.5,51.,60.));
#6544=CARTESIAN_POINT('Origin',(0.,9.,120.));
#6545=CARTESIAN_POINT('',(0.,9.,120.41));
#6546=CARTESIAN_POINT('Origin',(0.,9.,120.));
#6547=CARTESIAN_POINT('',(1.5,9.,120.41));
#6548=CARTESIAN_POINT('',(0.,9.,120.41));
#6549=CARTESIAN_POINT('Origin',(1.5,9.,120.));
#6550=CARTESIAN_POINT('Origin',(1.5,9.,120.));
#6551=CARTESIAN_POINT('Origin',(0.,9.,60.));
#6552=CARTESIAN_POINT('',(0.,9.,60.41));
#6553=CARTESIAN_POINT('Origin',(0.,9.,60.));
#6554=CARTESIAN_POINT('',(1.5,9.,60.41));
#6555=CARTESIAN_POINT('',(0.,9.,60.41));
#6556=CARTESIAN_POINT('Origin',(1.5,9.,60.));
#6557=CARTESIAN_POINT('Origin',(1.5,9.,60.));
#6558=CARTESIAN_POINT('Origin',(0.,51.,120.));
#6559=CARTESIAN_POINT('',(0.,51.,120.41));
#6560=CARTESIAN_POINT('Origin',(0.,51.,120.));
#6561=CARTESIAN_POINT('',(1.5,51.,120.41));
#6562=CARTESIAN_POINT('',(0.,51.,120.41));
#6563=CARTESIAN_POINT('Origin',(1.5,51.,120.));
#6564=CARTESIAN_POINT('Origin',(1.5,51.,120.));
#6565=CARTESIAN_POINT('Origin',(1.8,1.6,60.));
#6566=CARTESIAN_POINT('',(1.8,1.6,60.225));
#6567=CARTESIAN_POINT('Origin',(1.8,1.6,60.));
#6568=CARTESIAN_POINT('',(1.8,1.6,60.225));
#6569=CARTESIAN_POINT('Origin',(1.8,1.6,120.));
#6570=CARTESIAN_POINT('',(1.8,1.6,120.225));
#6571=CARTESIAN_POINT('Origin',(1.8,1.6,120.));
#6572=CARTESIAN_POINT('',(1.8,1.6,120.225));
#6573=CARTESIAN_POINT('Origin',(1.81,58.82,0.));
#6574=CARTESIAN_POINT('',(1.3,58.82,89.08));
#6575=CARTESIAN_POINT('',(1.8,58.82,89.08));
#6576=CARTESIAN_POINT('',(1.6825,58.82,89.08));
#6577=CARTESIAN_POINT('',(1.3,58.82,1.82));
#6578=CARTESIAN_POINT('',(1.3,58.82,0.));
#6579=CARTESIAN_POINT('',(1.8,58.82,1.82));
#6580=CARTESIAN_POINT('',(1.6825,58.82,1.82));
#6581=CARTESIAN_POINT('',(1.8,58.82,0.));
#6582=CARTESIAN_POINT('Origin',(1.81,58.82,0.));
#6583=CARTESIAN_POINT('',(1.3,58.82,178.18));
#6584=CARTESIAN_POINT('',(1.8,58.82,178.18));
#6585=CARTESIAN_POINT('',(1.6825,58.82,178.18));
#6586=CARTESIAN_POINT('',(1.3,58.82,90.92));
#6587=CARTESIAN_POINT('',(1.3,58.82,0.));
#6588=CARTESIAN_POINT('',(1.8,58.82,90.92));
#6589=CARTESIAN_POINT('',(1.6825,58.82,90.92));
#6590=CARTESIAN_POINT('',(1.8,58.82,0.));
#6591=CARTESIAN_POINT('Origin',(1.3,58.18,0.));
#6592=CARTESIAN_POINT('',(1.8,58.18,89.08));
#6593=CARTESIAN_POINT('',(1.3,58.18,89.08));
#6594=CARTESIAN_POINT('',(1.4275,58.18,89.08));
#6595=CARTESIAN_POINT('',(1.8,58.18,1.82));
#6596=CARTESIAN_POINT('',(1.8,58.18,0.));
#6597=CARTESIAN_POINT('',(1.3,58.18,1.82));
#6598=CARTESIAN_POINT('',(1.4275,58.18,1.82));
#6599=CARTESIAN_POINT('',(1.3,58.18,0.));
#6600=CARTESIAN_POINT('Origin',(1.3,58.18,0.));
#6601=CARTESIAN_POINT('',(1.8,58.18,178.18));
#6602=CARTESIAN_POINT('',(1.3,58.18,178.18));
#6603=CARTESIAN_POINT('',(1.4275,58.18,178.18));
#6604=CARTESIAN_POINT('',(1.8,58.18,90.92));
#6605=CARTESIAN_POINT('',(1.8,58.18,0.));
#6606=CARTESIAN_POINT('',(1.3,58.18,90.92));
#6607=CARTESIAN_POINT('',(1.4275,58.18,90.92));
#6608=CARTESIAN_POINT('',(1.3,58.18,0.));
#6609=CARTESIAN_POINT('Origin',(1.3,60.,178.18));
#6610=CARTESIAN_POINT('',(1.3,60.,178.18));
#6611=CARTESIAN_POINT('',(1.3,60.,178.18));
#6612=CARTESIAN_POINT('',(1.3,60.,180.));
#6613=CARTESIAN_POINT('',(1.3,60.,89.09));
#6614=CARTESIAN_POINT('',(1.3,0.,180.));
#6615=CARTESIAN_POINT('',(1.3,45.,180.));
#6616=CARTESIAN_POINT('',(1.3,0.,178.18));
#6617=CARTESIAN_POINT('',(1.3,0.,89.09));
#6618=CARTESIAN_POINT('',(1.3,60.,178.18));
#6619=CARTESIAN_POINT('',(1.3,0.,90.92));
#6620=CARTESIAN_POINT('',(1.3,60.,90.92));
#6621=CARTESIAN_POINT('',(1.3,0.,89.08));
#6622=CARTESIAN_POINT('',(1.3,0.,44.54));
#6623=CARTESIAN_POINT('',(1.3,60.,89.08));
#6624=CARTESIAN_POINT('',(1.3,0.,1.82));
#6625=CARTESIAN_POINT('',(1.3,60.,1.82));
#6626=CARTESIAN_POINT('',(1.3,0.,0.));
#6627=CARTESIAN_POINT('',(1.3,0.,0.));
#6628=CARTESIAN_POINT('',(1.3,60.,0.));
#6629=CARTESIAN_POINT('',(1.3,45.,0.));
#6630=CARTESIAN_POINT('',(1.3,60.,1.82));
#6631=CARTESIAN_POINT('',(1.3,60.,0.));
#6632=CARTESIAN_POINT('',(1.3,60.,1.82));
#6633=CARTESIAN_POINT('',(1.3,60.,89.08));
#6634=CARTESIAN_POINT('',(1.3,60.,89.08));
#6635=CARTESIAN_POINT('',(1.3,60.,90.92));
#6636=CARTESIAN_POINT('',(1.3,60.,44.54));
#6637=CARTESIAN_POINT('',(1.3,60.,90.92));
#6638=CARTESIAN_POINT('Origin',(1.555,30.,178.18));
#6639=CARTESIAN_POINT('',(1.8,0.,178.18));
#6640=CARTESIAN_POINT('',(0.7775,0.,178.18));
#6641=CARTESIAN_POINT('',(1.8,15.,178.18));
#6642=CARTESIAN_POINT('Origin',(1.555,30.,178.18));
#6643=CARTESIAN_POINT('',(1.8,60.,178.18));
#6644=CARTESIAN_POINT('',(1.8,15.,178.18));
#6645=CARTESIAN_POINT('',(1.6775,60.,178.18));
#6646=CARTESIAN_POINT('Origin',(1.8,0.,0.));
#6647=CARTESIAN_POINT('',(1.8,0.,90.92));
#6648=CARTESIAN_POINT('',(1.8,0.,0.));
#6649=CARTESIAN_POINT('',(1.8,15.,90.92));
#6650=CARTESIAN_POINT('Origin',(1.8,0.,0.));
#6651=CARTESIAN_POINT('',(1.8,60.,90.92));
#6652=CARTESIAN_POINT('',(1.8,15.,90.92));
#6653=CARTESIAN_POINT('',(1.8,60.,0.));
#6654=CARTESIAN_POINT('Origin',(1.555,30.,90.92));
#6655=CARTESIAN_POINT('',(0.7775,0.,90.92));
#6656=CARTESIAN_POINT('Origin',(1.555,30.,90.92));
#6657=CARTESIAN_POINT('',(1.6775,60.,90.92));
#6658=CARTESIAN_POINT('Origin',(1.555,30.,89.08));
#6659=CARTESIAN_POINT('',(1.8,0.,89.08));
#6660=CARTESIAN_POINT('',(0.7775,0.,89.08));
#6661=CARTESIAN_POINT('',(1.8,15.,89.08));
#6662=CARTESIAN_POINT('Origin',(1.555,30.,89.08));
#6663=CARTESIAN_POINT('',(1.8,60.,89.08));
#6664=CARTESIAN_POINT('',(1.8,15.,89.08));
#6665=CARTESIAN_POINT('',(1.6775,60.,89.08));
#6666=CARTESIAN_POINT('Origin',(1.8,0.,0.));
#6667=CARTESIAN_POINT('',(1.8,0.,1.82));
#6668=CARTESIAN_POINT('',(1.8,0.,0.));
#6669=CARTESIAN_POINT('',(1.8,15.,1.82));
#6670=CARTESIAN_POINT('Origin',(1.8,0.,0.));
#6671=CARTESIAN_POINT('',(1.8,60.,1.82));
#6672=CARTESIAN_POINT('',(1.8,15.,1.82));
#6673=CARTESIAN_POINT('',(1.8,60.,0.));
#6674=CARTESIAN_POINT('Origin',(1.555,30.,1.82));
#6675=CARTESIAN_POINT('',(0.7775,0.,1.82));
#6676=CARTESIAN_POINT('Origin',(1.555,30.,1.82));
#6677=CARTESIAN_POINT('',(1.6775,60.,1.82));
#6678=CARTESIAN_POINT('Origin',(1.8,60.,0.));
#6679=CARTESIAN_POINT('',(0.,60.,0.));
#6680=CARTESIAN_POINT('',(1.8,60.,0.));
#6681=CARTESIAN_POINT('',(0.,60.,180.));
#6682=CARTESIAN_POINT('',(0.,60.,0.));
#6683=CARTESIAN_POINT('',(1.8,60.,180.));
#6684=CARTESIAN_POINT('Origin',(0.9,30.,0.));
#6685=CARTESIAN_POINT('',(0.,0.,0.));
#6686=CARTESIAN_POINT('',(0.,0.,0.));
#6687=CARTESIAN_POINT('',(0.,60.,0.));
#6688=CARTESIAN_POINT('Origin',(0.,0.,0.));
#6689=CARTESIAN_POINT('',(0.,0.,180.));
#6690=CARTESIAN_POINT('',(0.,0.,180.));
#6691=CARTESIAN_POINT('',(0.,0.,0.));
#6692=CARTESIAN_POINT('Origin',(0.,60.,0.));
#6693=CARTESIAN_POINT('',(0.,60.,180.));
#6694=CARTESIAN_POINT('Origin',(0.9,30.,180.));
#12937=UNCERTAINTY_MEASURE_WITH_UNIT(LENGTH_MEASURE(0.001),#12964,
'DISTANCE_ACCURACY_VALUE',
'Maximum model space distance between geometric entities at asserted c
onnectivities');
#12949=UNCERTAINTY_MEASURE_WITH_UNIT(LENGTH_MEASURE(0.001),#12964,
'DISTANCE_ACCURACY_VALUE',
'Maximum model space distance between geometric entities at asserted c
onnectivities');
#12951=(
GEOMETRIC_REPRESENTATION_CONTEXT(3)
GLOBAL_UNCERTAINTY_ASSIGNED_CONTEXT((#12937))
GLOBAL_UNIT_ASSIGNED_CONTEXT((#12964,#12966,#12967))
REPRESENTATION_CONTEXT('','3D')
);
#12963=(
GEOMETRIC_REPRESENTATION_CONTEXT(3)
GLOBAL_UNCERTAINTY_ASSIGNED_CONTEXT((#12949))
GLOBAL_UNIT_ASSIGNED_CONTEXT((#12964,#12966,#12967))
REPRESENTATION_CONTEXT('','3D')
);
#12964=(
LENGTH_UNIT()
NAMED_UNIT(*)
SI_UNIT(.CENTI.,.METRE.)
);
#12966=(
NAMED_UNIT(*)
PLANE_ANGLE_UNIT()
SI_UNIT($,.RADIAN.)
);
#12967=(
NAMED_UNIT(*)
SI_UNIT($,.STERADIAN.)
SOLID_ANGLE_UNIT()
);
#12969=SHAPE_DEFINITION_REPRESENTATION(#12982,#13035);
#12982=PRODUCT_DEFINITION_SHAPE('',$,#13049);
#13035=SHAPE_REPRESENTATION('',(#4955),#12951);
#13047=PRODUCT_DEFINITION_CONTEXT('part definition',#13088,'design');
#13049=PRODUCT_DEFINITION('Side panel with hardware clearance',
'Side panel with hardware clearance',#13062,#13047);
#13062=PRODUCT_DEFINITION_FORMATION('',$,#13091);
#13088=APPLICATION_CONTEXT(
'Core Data for Automotive Mechanical Design Process');
#13089=PRODUCT_CONTEXT('part definition',#13088,'mechanical');
#13091=PRODUCT('Side panel with hardware clearance',
'Side panel with hardware clearance',$,(#13089));
#13104=PRESENTATION_STYLE_ASSIGNMENT((#13117));
#13117=SURFACE_STYLE_USAGE(.BOTH.,#13130);
#13130=SURFACE_SIDE_STYLE('',(#13143));
#13143=SURFACE_STYLE_FILL_AREA(#13156);
#13156=FILL_AREA_STYLE('Side panel with hardware clearance finish',(#13169));
#13169=FILL_AREA_STYLE_COLOUR(
'Side panel with hardware clearance finish',#13182);
#13182=COLOUR_RGB('Side panel with hardware clearance finish',0.0941176470588235,
0.231372549019608,0.431372549019608);
ENDSEC;
END-ISO-10303-21;
